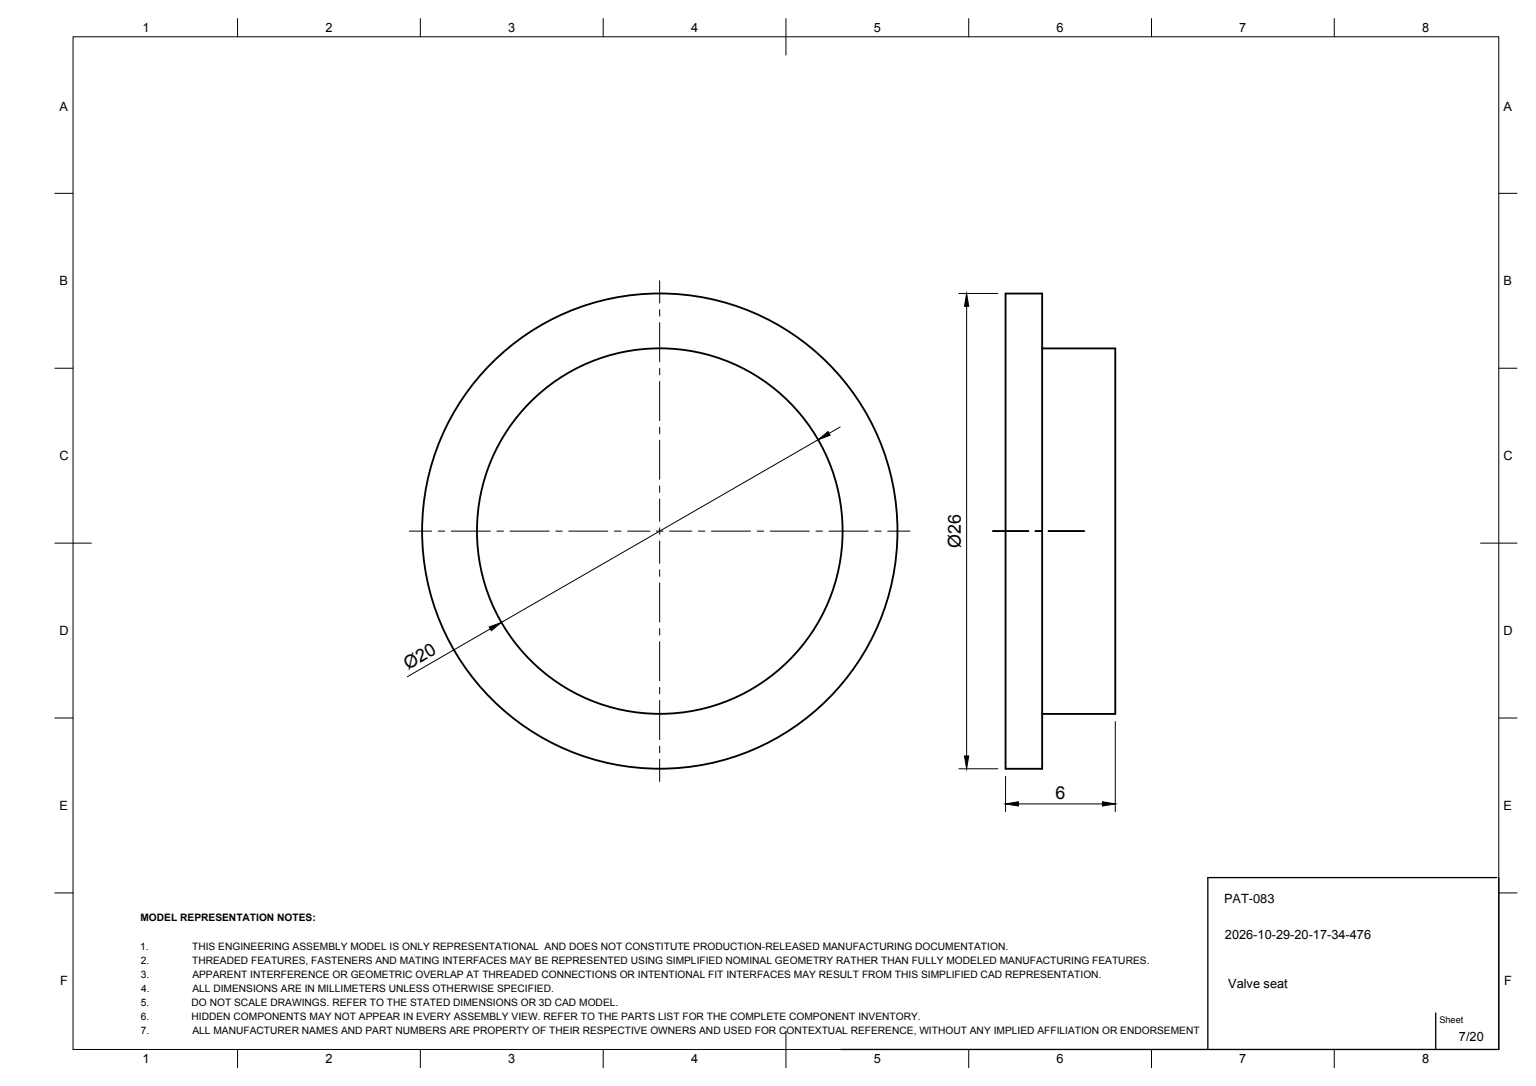
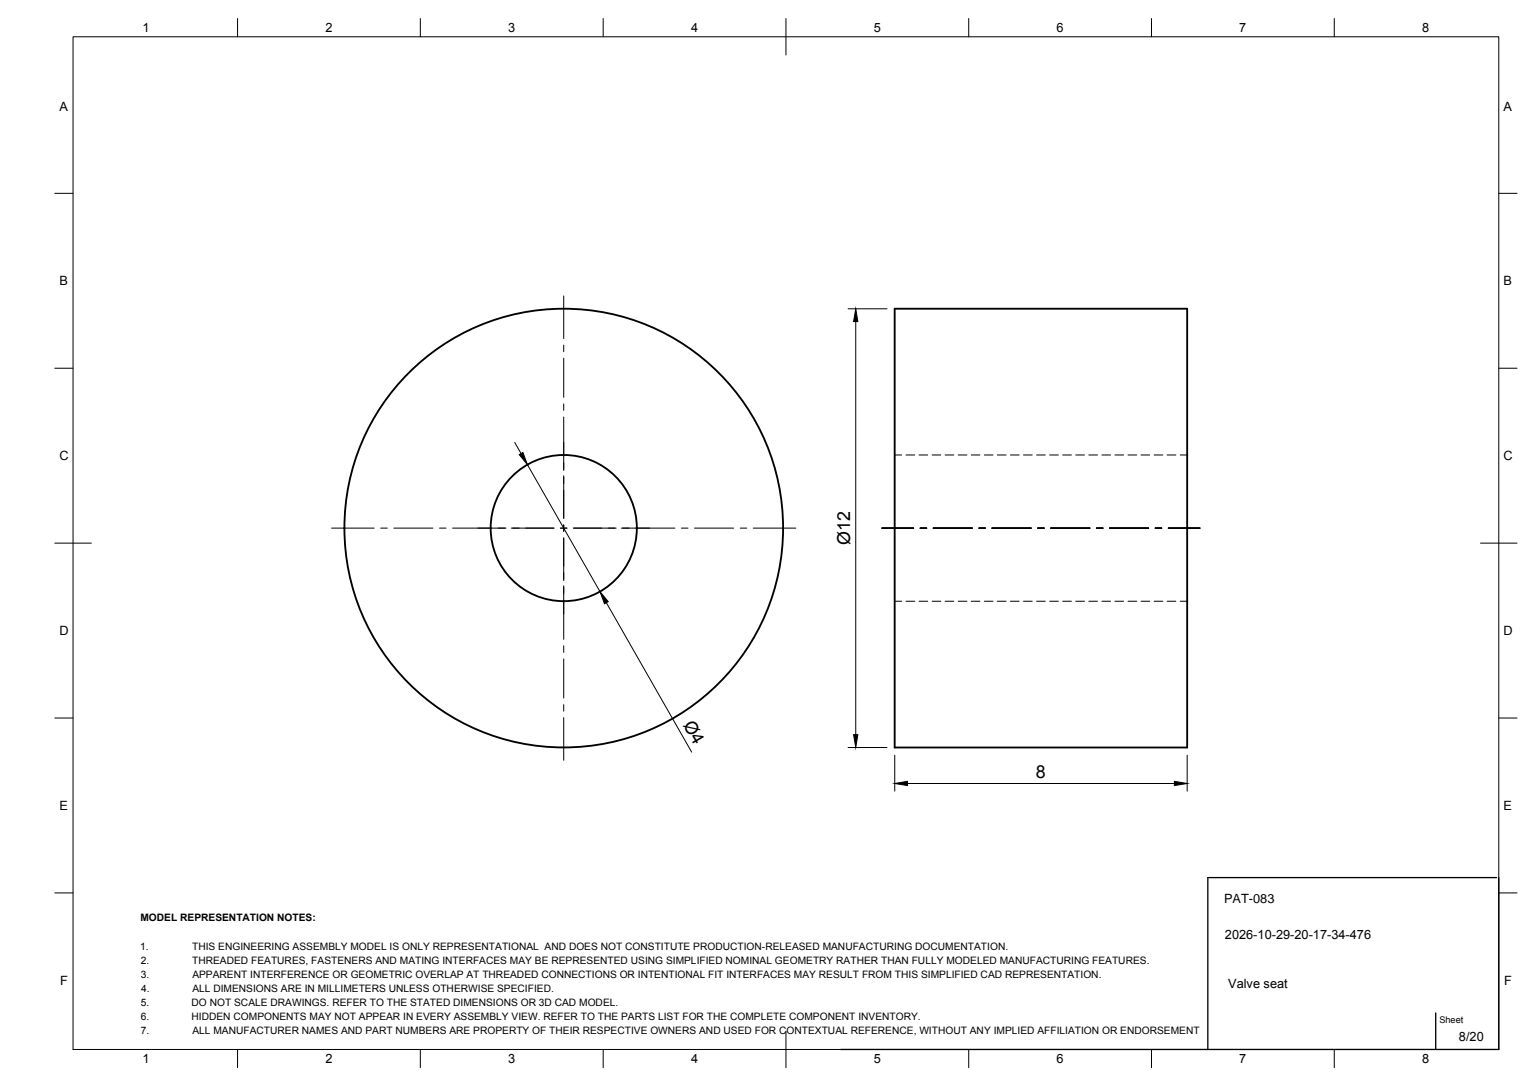
ISO-10303-21;
HEADER;
/* Generated by software containing ST-Developer
 * from STEP Tools, Inc. (www.steptools.com) 
 */

FILE_DESCRIPTION(
/* description */ ('PAT-083'),
/* implementation_level */ '2;1');

FILE_NAME(
/* name */ 'Valve seat.step',
/* time_stamp */ '2026-10-29T20:18:00-07:00',
/* author */ (''),
/* organization */ (''),
/* preprocessor_version */ 'ST-DEVELOPER v20.2',
/* originating_system */ 'Autodesk Translation Framework v15.17.0.0',
/* authorisation */ '');

FILE_SCHEMA (('AUTOMOTIVE_DESIGN { 1 0 10303 214 3 1 1 }'));
ENDSEC;

DATA;
#10=MECHANICAL_DESIGN_GEOMETRIC_PRESENTATION_REPRESENTATION('',(#234),#8428);
#186=SHAPE_REPRESENTATION_RELATIONSHIP('SRR','None',#8520,#210);
#210=ADVANCED_BREP_SHAPE_REPRESENTATION('',(#258),#8409);
#234=STYLED_ITEM('',(#8719),#258);
#258=MANIFOLD_SOLID_BREP('Body1',#3680);
#298=FACE_BOUND('',#815,.T.);
#299=FACE_BOUND('',#817,.T.);
#393=PLANE('',#4084);
#394=PLANE('',#4085);
#556=FACE_OUTER_BOUND('',#812,.T.);
#557=FACE_OUTER_BOUND('',#813,.T.);
#558=FACE_OUTER_BOUND('',#814,.T.);
#559=FACE_OUTER_BOUND('',#816,.T.);
#812=EDGE_LOOP('',(#2696,#2697,#2698,#2699));
#813=EDGE_LOOP('',(#2700,#2701,#2702,#2703));
#814=EDGE_LOOP('',(#2704));
#815=EDGE_LOOP('',(#2705));
#816=EDGE_LOOP('',(#2706));
#817=EDGE_LOOP('',(#2707));
#1108=LINE('',#6024,#1352);
#1109=LINE('',#6030,#1353);
#1352=VECTOR('',#4730,0.2);
#1353=VECTOR('',#4737,0.6);
#1574=CIRCLE('',#4079,0.2);
#1575=CIRCLE('',#4080,0.2);
#1576=CIRCLE('',#4082,0.6);
#1577=CIRCLE('',#4083,0.6);
#1787=VERTEX_POINT('',#6021);
#1788=VERTEX_POINT('',#6023);
#1789=VERTEX_POINT('',#6027);
#1790=VERTEX_POINT('',#6029);
#2124=EDGE_CURVE('',#1787,#1787,#1574,.T.);
#2125=EDGE_CURVE('',#1787,#1788,#1108,.T.);
#2126=EDGE_CURVE('',#1788,#1788,#1575,.T.);
#2127=EDGE_CURVE('',#1789,#1789,#1576,.T.);
#2128=EDGE_CURVE('',#1789,#1790,#1109,.T.);
#2129=EDGE_CURVE('',#1790,#1790,#1577,.T.);
#2696=ORIENTED_EDGE('',*,*,#2124,.F.);
#2697=ORIENTED_EDGE('',*,*,#2125,.T.);
#2698=ORIENTED_EDGE('',*,*,#2126,.T.);
#2699=ORIENTED_EDGE('',*,*,#2125,.F.);
#2700=ORIENTED_EDGE('',*,*,#2127,.F.);
#2701=ORIENTED_EDGE('',*,*,#2128,.T.);
#2702=ORIENTED_EDGE('',*,*,#2129,.T.);
#2703=ORIENTED_EDGE('',*,*,#2128,.F.);
#2704=ORIENTED_EDGE('',*,*,#2127,.T.);
#2705=ORIENTED_EDGE('',*,*,#2124,.T.);
#2706=ORIENTED_EDGE('',*,*,#2129,.F.);
#2707=ORIENTED_EDGE('',*,*,#2126,.F.);
#3388=CYLINDRICAL_SURFACE('',#4078,0.2);
#3389=CYLINDRICAL_SURFACE('',#4081,0.6);
#3503=ADVANCED_FACE('',(#556),#3388,.F.);
#3504=ADVANCED_FACE('',(#557),#3389,.T.);
#3505=ADVANCED_FACE('',(#558,#298),#393,.T.);
#3506=ADVANCED_FACE('',(#559,#299),#394,.F.);
#3680=CLOSED_SHELL('',(#3503,#3504,#3505,#3506));
#4077=AXIS2_PLACEMENT_3D('',#6019,#4724,#4725);
#4078=AXIS2_PLACEMENT_3D('',#6020,#4726,#4727);
#4079=AXIS2_PLACEMENT_3D('',#6022,#4728,#4729);
#4080=AXIS2_PLACEMENT_3D('',#6025,#4731,#4732);
#4081=AXIS2_PLACEMENT_3D('',#6026,#4733,#4734);
#4082=AXIS2_PLACEMENT_3D('',#6028,#4735,#4736);
#4083=AXIS2_PLACEMENT_3D('',#6031,#4738,#4739);
#4084=AXIS2_PLACEMENT_3D('',#6032,#4740,#4741);
#4085=AXIS2_PLACEMENT_3D('',#6033,#4742,#4743);
#4724=DIRECTION('axis',(0.,0.,1.));
#4725=DIRECTION('refdir',(1.,0.,0.));
#4726=DIRECTION('center_axis',(0.,0.,1.));
#4727=DIRECTION('ref_axis',(1.,0.,0.));
#4728=DIRECTION('center_axis',(0.,0.,-1.));
#4729=DIRECTION('ref_axis',(1.,0.,0.));
#4730=DIRECTION('',(0.,0.,-1.));
#4731=DIRECTION('center_axis',(0.,0.,-1.));
#4732=DIRECTION('ref_axis',(1.,0.,0.));
#4733=DIRECTION('center_axis',(0.,0.,1.));
#4734=DIRECTION('ref_axis',(1.,0.,0.));
#4735=DIRECTION('center_axis',(0.,0.,1.));
#4736=DIRECTION('ref_axis',(1.,0.,0.));
#4737=DIRECTION('',(0.,0.,-1.));
#4738=DIRECTION('center_axis',(0.,0.,1.));
#4739=DIRECTION('ref_axis',(1.,0.,0.));
#4740=DIRECTION('center_axis',(0.,0.,1.));
#4741=DIRECTION('ref_axis',(1.,0.,0.));
#4742=DIRECTION('center_axis',(0.,0.,1.));
#4743=DIRECTION('ref_axis',(1.,0.,0.));
#6019=CARTESIAN_POINT('',(0.,0.,0.));
#6020=CARTESIAN_POINT('Origin',(0.,0.,2.4));
#6021=CARTESIAN_POINT('',(-0.2,-2.44929359829471E-17,3.2));
#6022=CARTESIAN_POINT('Origin',(0.,0.,3.2));
#6023=CARTESIAN_POINT('',(-0.2,-2.44929359829471E-17,2.4));
#6024=CARTESIAN_POINT('',(-0.2,-2.44929359829471E-17,2.4));
#6025=CARTESIAN_POINT('Origin',(0.,0.,2.4));
#6026=CARTESIAN_POINT('Origin',(0.,0.,2.4));
#6027=CARTESIAN_POINT('',(-0.6,-7.34788079488412E-17,3.2));
#6028=CARTESIAN_POINT('Origin',(0.,0.,3.2));
#6029=CARTESIAN_POINT('',(-0.6,-7.34788079488412E-17,2.4));
#6030=CARTESIAN_POINT('',(-0.6,-7.34788079488412E-17,2.4));
#6031=CARTESIAN_POINT('Origin',(0.,0.,2.4));
#6032=CARTESIAN_POINT('Origin',(0.,0.,3.2));
#6033=CARTESIAN_POINT('Origin',(0.,0.,2.4));
#8383=UNCERTAINTY_MEASURE_WITH_UNIT(LENGTH_MEASURE(0.001),#8429,
'DISTANCE_ACCURACY_VALUE',
'Maximum model space distance between geometric entities at asserted c
onnectivities');
#8402=UNCERTAINTY_MEASURE_WITH_UNIT(LENGTH_MEASURE(0.001),#8429,
'DISTANCE_ACCURACY_VALUE',
'Maximum model space distance between geometric entities at asserted c
onnectivities');
#8409=(
GEOMETRIC_REPRESENTATION_CONTEXT(3)
GLOBAL_UNCERTAINTY_ASSIGNED_CONTEXT((#8383))
GLOBAL_UNIT_ASSIGNED_CONTEXT((#8429,#8431,#8432))
REPRESENTATION_CONTEXT('','3D')
);
#8428=(
GEOMETRIC_REPRESENTATION_CONTEXT(3)
GLOBAL_UNCERTAINTY_ASSIGNED_CONTEXT((#8402))
GLOBAL_UNIT_ASSIGNED_CONTEXT((#8429,#8431,#8432))
REPRESENTATION_CONTEXT('','3D')
);
#8429=(
LENGTH_UNIT()
NAMED_UNIT(*)
SI_UNIT(.CENTI.,.METRE.)
);
#8431=(
NAMED_UNIT(*)
PLANE_ANGLE_UNIT()
SI_UNIT($,.RADIAN.)
);
#8432=(
NAMED_UNIT(*)
SI_UNIT($,.STERADIAN.)
SOLID_ANGLE_UNIT()
);
#8439=SHAPE_DEFINITION_REPRESENTATION(#8464,#8520);
#8464=PRODUCT_DEFINITION_SHAPE('',$,#8546);
#8520=SHAPE_REPRESENTATION('',(#4077),#8409);
#8539=PRODUCT_DEFINITION_CONTEXT('part definition',#8616,'design');
#8546=PRODUCT_DEFINITION('Valve seat','Valve seat',#8571,
#8539);
#8571=PRODUCT_DEFINITION_FORMATION('',$,#8624);
#8616=APPLICATION_CONTEXT(
'Core Data for Automotive Mechanical Design Process');
#8617=PRODUCT_CONTEXT('part definition',#8616,'mechanical');
#8624=PRODUCT('Valve seat','Valve seat','Valve seat',(#8617));
#8713=COLOUR_RGB('Off White',0.89,0.88,0.83);
#8714=FILL_AREA_STYLE_COLOUR('',#8713);
#8715=FILL_AREA_STYLE('',(#8714));
#8716=SURFACE_STYLE_FILL_AREA(#8715);
#8717=SURFACE_SIDE_STYLE('',(#8716));
#8718=SURFACE_STYLE_USAGE(.BOTH.,#8717);
#8719=PRESENTATION_STYLE_ASSIGNMENT((#8718));
ENDSEC;
END-ISO-10303-21;
